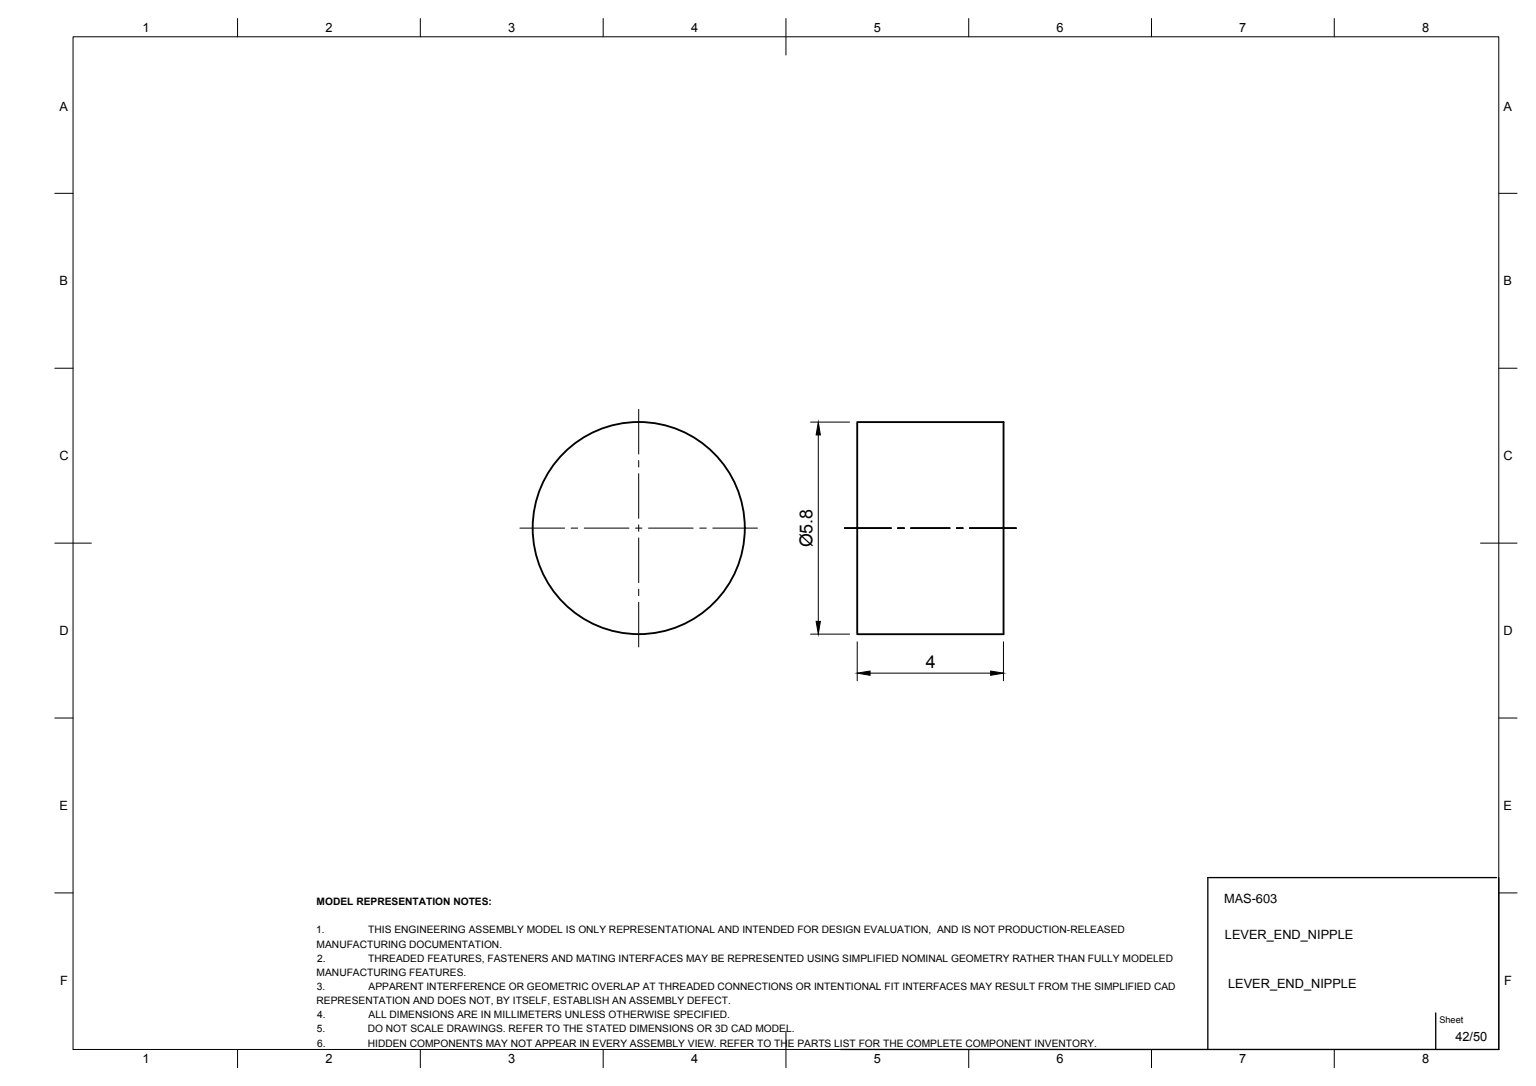
ISO-10303-21;
HEADER;
FILE_DESCRIPTION((''),'2;1');
FILE_NAME('LEVER_END_NIPPLE.step','2026-10-01T22:06:14-07:00',(''),(''),'','','');
FILE_SCHEMA (('AUTOMOTIVE_DESIGN { 1 0 10303 214 3 1 1 }'));
ENDSEC;
DATA;
#10=MECHANICAL_DESIGN_GEOMETRIC_PRESENTATION_REPRESENTATION('',(#1016),#50440);
#922=SHAPE_REPRESENTATION_RELATIONSHIP('SRR','None',#50655,#967) ;
#967=ADVANCED_BREP_SHAPE_REPRESENTATION('',(#1070),#50424) ;
#1016=STYLED_ITEM('',(#50887),#1070) ;
#1070=MANIFOLD_SOLID_BREP('LEVER_END_NIPPLE',#28692) ;
#2242=PLANE('',#31067) ;
#2243=PLANE('',#31068) ;
#3472=FACE_OUTER_BOUND('',#5293,.T.) ;
#3473=FACE_OUTER_BOUND('',#5294,.T.) ;
#3474=FACE_OUTER_BOUND('',#5295,.T.) ;
#5293=EDGE_LOOP('',(#24289,#24290,#24291,#24292)) ;
#5294=EDGE_LOOP('',(#24293)) ;
#5295=EDGE_LOOP('',(#24294)) ;
#7900=LINE('',#47516,#10372) ;
#10372=VECTOR('',#38257,0.29) ;
#11293=CIRCLE('',#31065,0.29) ;
#11294=CIRCLE('',#31066,0.29) ;
#13751=VERTEX_POINT('',#47513) ;
#13752=VERTEX_POINT('',#47515) ;
#17410=EDGE_CURVE('',#13751,#13751,#11293,.T.) ;
#17411=EDGE_CURVE('',#13751,#13752,#7900,.T.) ;
#17412=EDGE_CURVE('',#13752,#13752,#11294,.T.) ;
#24289=ORIENTED_EDGE('',*,*,#17410,.F.) ;
#24290=ORIENTED_EDGE('',*,*,#17411,.T.) ;
#24291=ORIENTED_EDGE('',*,*,#17412,.F.) ;
#24292=ORIENTED_EDGE('',*,*,#17411,.F.) ;
#24293=ORIENTED_EDGE('',*,*,#17412,.T.) ;
#24294=ORIENTED_EDGE('',*,*,#17410,.T.) ;
#26894=CYLINDRICAL_SURFACE('',#31064,0.29) ;
#28207=ADVANCED_FACE('',(#3472),#26894,.T.) ;
#28208=ADVANCED_FACE('',(#3473),#2242,.T.) ;
#28209=ADVANCED_FACE('',(#3474),#2243,.T.) ;
#28692=CLOSED_SHELL('',(#28207,#28208,#28209)) ;
#31063=AXIS2_PLACEMENT_3D('',#47511,#38251,#38252) ;
#31064=AXIS2_PLACEMENT_3D('',#47512,#38253,#38254) ;
#31065=AXIS2_PLACEMENT_3D('',#47514,#38255,#38256) ;
#31066=AXIS2_PLACEMENT_3D('',#47517,#38258,#38259) ;
#31067=AXIS2_PLACEMENT_3D('',#47518,#38260,#38261) ;
#31068=AXIS2_PLACEMENT_3D('',#47519,#38262,#38263) ;
#38251=DIRECTION('axis',(0.,0.,1.)) ;
#38252=DIRECTION('refdir',(1.,0.,0.)) ;
#38253=DIRECTION('center_axis',(0.,0.,1.)) ;
#38254=DIRECTION('ref_axis',(1.,0.,0.)) ;
#38255=DIRECTION('center_axis',(0.,0.,1.)) ;
#38256=DIRECTION('ref_axis',(1.,0.,0.)) ;
#38257=DIRECTION('',(0.,0.,-1.)) ;
#38258=DIRECTION('center_axis',(0.,0.,-1.)) ;
#38259=DIRECTION('ref_axis',(1.,0.,0.)) ;
#38260=DIRECTION('center_axis',(0.,0.,-1.)) ;
#38261=DIRECTION('ref_axis',(-1.,0.,0.)) ;
#38262=DIRECTION('center_axis',(0.,0.,1.)) ;
#38263=DIRECTION('ref_axis',(1.,0.,0.)) ;
#47511=CARTESIAN_POINT('',(0.,0.,0.)) ;
#47512=CARTESIAN_POINT('Origin',(-53.,19.,89.6)) ;
#47513=CARTESIAN_POINT('',(-53.29,19.,89.8)) ;
#47514=CARTESIAN_POINT('Origin',(-53.,19.,89.8)) ;
#47515=CARTESIAN_POINT('',(-53.29,19.,89.4)) ;
#47516=CARTESIAN_POINT('',(-53.29,19.,89.6)) ;
#47517=CARTESIAN_POINT('Origin',(-53.,19.,89.4)) ;
#47518=CARTESIAN_POINT('Origin',(-53.,19.,89.4)) ;
#47519=CARTESIAN_POINT('Origin',(-53.,19.,89.8)) ;
#50371=UNCERTAINTY_MEASURE_WITH_UNIT(LENGTH_MEASURE(0.001),#50441,
'DISTANCE_ACCURACY_VALUE',
'Maximum model space distance between geometric entities at asserted c
onnectivities') ;
#50387=UNCERTAINTY_MEASURE_WITH_UNIT(LENGTH_MEASURE(0.001),#50441,
'DISTANCE_ACCURACY_VALUE',
'Maximum model space distance between geometric entities at asserted c
onnectivities') ;
#50424=(
GEOMETRIC_REPRESENTATION_CONTEXT(3)
GLOBAL_UNCERTAINTY_ASSIGNED_CONTEXT((#50371))
GLOBAL_UNIT_ASSIGNED_CONTEXT((#50441,#50443,#50444))
REPRESENTATION_CONTEXT('','3D')
) ;
#50440=(
GEOMETRIC_REPRESENTATION_CONTEXT(3)
GLOBAL_UNCERTAINTY_ASSIGNED_CONTEXT((#50387))
GLOBAL_UNIT_ASSIGNED_CONTEXT((#50441,#50443,#50444))
REPRESENTATION_CONTEXT('','3D')
) ;
#50441=(
LENGTH_UNIT()
NAMED_UNIT(*)
SI_UNIT(.CENTI.,.METRE.)
) ;
#50443=(
NAMED_UNIT(*)
PLANE_ANGLE_UNIT()
SI_UNIT($,.RADIAN.)
) ;
#50444=(
NAMED_UNIT(*)
SI_UNIT($,.STERADIAN.)
SOLID_ANGLE_UNIT()
) ;
#50481=SHAPE_DEFINITION_REPRESENTATION(#50557,#50655) ;
#50557=PRODUCT_DEFINITION_SHAPE('',$,#50708) ;
#50655=SHAPE_REPRESENTATION('',(#31063),#50424) ;
#50671=PRODUCT_DEFINITION_CONTEXT('part definition',#50829,'design') ;
#50708=PRODUCT_DEFINITION('LEVER_END_NIPPLE','LEVER_END_NIPPLE',
#50760,#50671) ;
#50760=PRODUCT_DEFINITION_FORMATION('',$,#50867) ;
#50829=APPLICATION_CONTEXT(
'Core Data for Automotive Mechanical Design Process') ;
#50830=PRODUCT_CONTEXT('part definition',#50829,'mechanical') ;
#50867=PRODUCT('LEVER_END_NIPPLE','LEVER_END_NIPPLE',$,(#50830)) ;
#50887=PRESENTATION_STYLE_ASSIGNMENT((#50894)) ;
#50894=SURFACE_STYLE_USAGE(.BOTH.,#50901) ;
#50901=SURFACE_SIDE_STYLE('',(#50908)) ;
#50908=SURFACE_STYLE_FILL_AREA(#50915) ;
#50915=FILL_AREA_STYLE('Brass - Polished',(#50922)) ;
#50922=FILL_AREA_STYLE_COLOUR('Brass - Polished',#50929) ;
#50929=COLOUR_RGB('Brass - Polished', 0.66274510, 0.83137255, 0.94901961) ;
ENDSEC;
END-ISO-10303-21;
